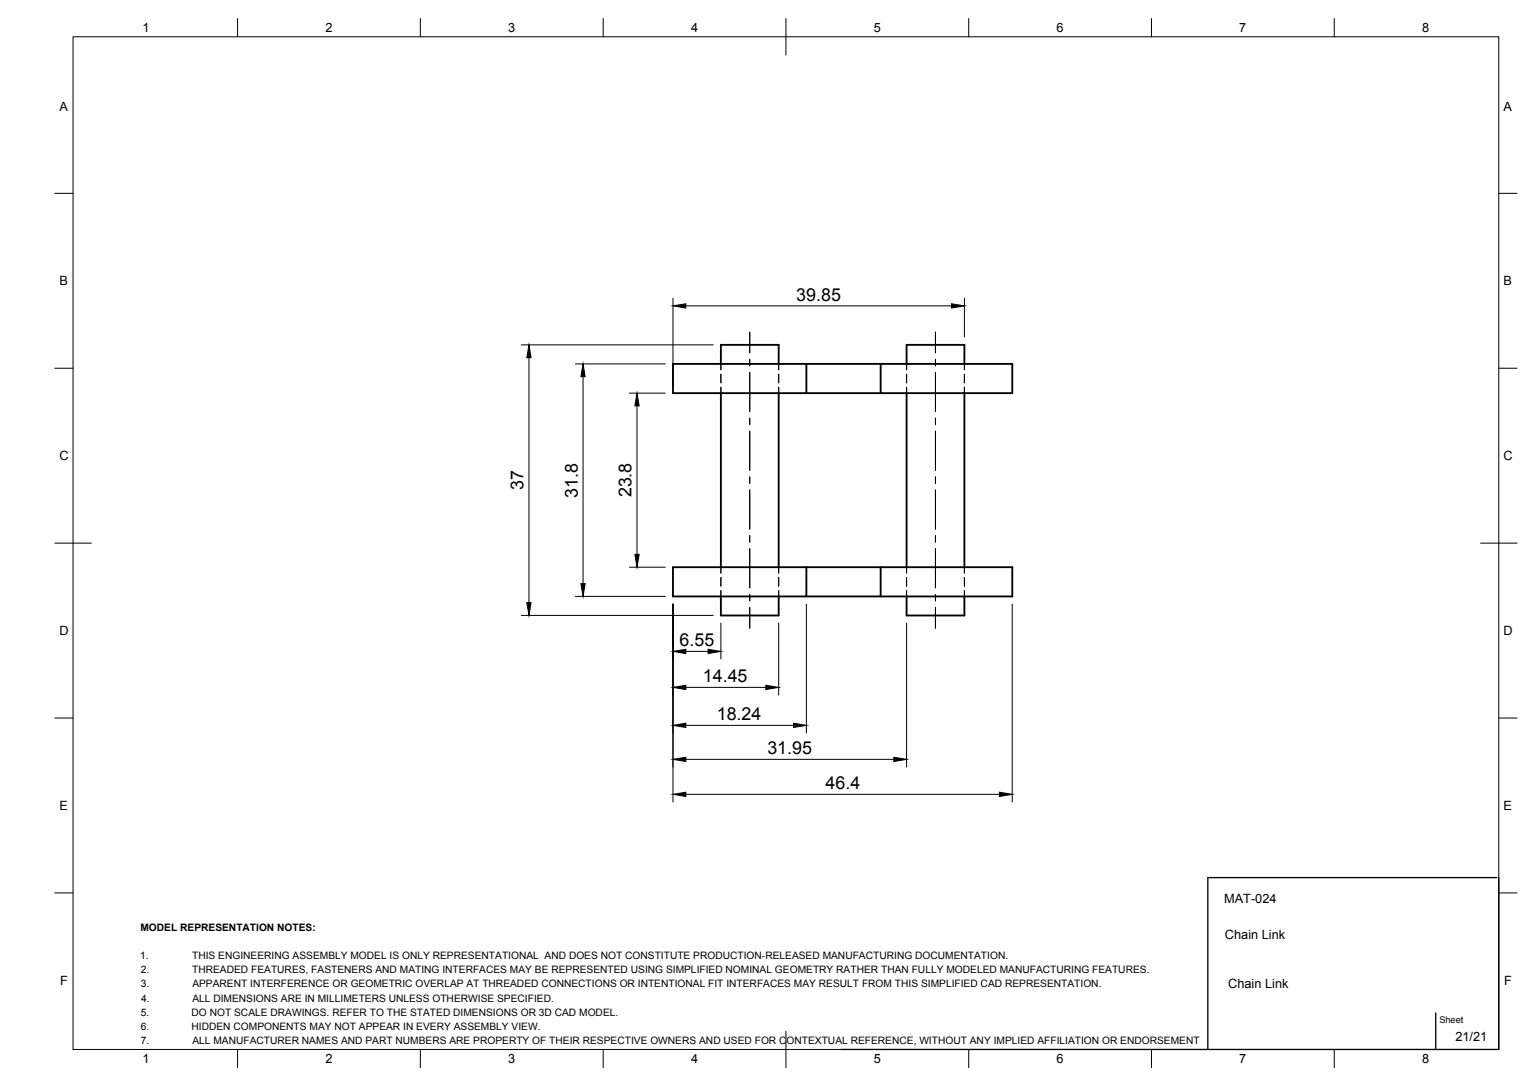
ISO-10303-21;
HEADER;
/* Generated by software containing ST-Developer
 * from STEP Tools, Inc. (www.steptools.com) 
 */

FILE_DESCRIPTION(
/* description */ ('STEP AP214'),
/* implementation_level */ '2;1');

FILE_NAME(
/* name */ 'Chain Link.step',
/* time_stamp */ '2026-11-14T06:34:07-08:00',
/* author */ (''),
/* organization */ (''),
/* preprocessor_version */ 'ST-DEVELOPER v20.2',
/* originating_system */ 'Autodesk Translation Framework v15.17.0.0',
/* authorisation */ '');

FILE_SCHEMA (('AUTOMOTIVE_DESIGN { 1 0 10303 214 3 1 1 }'));
ENDSEC;

DATA;
#10=MECHANICAL_DESIGN_GEOMETRIC_PRESENTATION_REPRESENTATION('',(#7282,#7283,#7284,#7285),#310623);
#7228=SHAPE_REPRESENTATION_RELATIONSHIP('SRR','None',#310901,#7245);
#7245=ADVANCED_BREP_SHAPE_REPRESENTATION('',(#7350,#7351,#7352,#7353),#310610);
#7282=STYLED_ITEM('',(#311007),#7350);
#7283=STYLED_ITEM('',(#311007),#7351);
#7284=STYLED_ITEM('',(#311007),#7352);
#7285=STYLED_ITEM('',(#311007),#7353);
#7350=MANIFOLD_SOLID_BREP('Body1',#93732);
#7351=MANIFOLD_SOLID_BREP('Body2',#93733);
#7352=MANIFOLD_SOLID_BREP('Body3',#93734);
#7353=MANIFOLD_SOLID_BREP('Body4',#93735);
#7630=FACE_BOUND('',#19915,.T.);
#7631=FACE_BOUND('',#19916,.T.);
#7632=FACE_BOUND('',#19918,.T.);
#7633=FACE_BOUND('',#19919,.T.);
#7634=FACE_BOUND('',#19924,.T.);
#7635=FACE_BOUND('',#19925,.T.);
#7636=FACE_BOUND('',#19927,.T.);
#7637=FACE_BOUND('',#19928,.T.);
#8541=PLANE('',#103942);
#8542=PLANE('',#103943);
#8543=PLANE('',#103953);
#8544=PLANE('',#103957);
#8545=PLANE('',#103967);
#8546=PLANE('',#103968);
#8547=PLANE('',#103972);
#8548=PLANE('',#103973);
#13930=FACE_OUTER_BOUND('',#19908,.T.);
#13931=FACE_OUTER_BOUND('',#19909,.T.);
#13932=FACE_OUTER_BOUND('',#19910,.T.);
#13933=FACE_OUTER_BOUND('',#19911,.T.);
#13934=FACE_OUTER_BOUND('',#19912,.T.);
#13935=FACE_OUTER_BOUND('',#19913,.T.);
#13936=FACE_OUTER_BOUND('',#19914,.T.);
#13937=FACE_OUTER_BOUND('',#19917,.T.);
#13938=FACE_OUTER_BOUND('',#19920,.T.);
#13939=FACE_OUTER_BOUND('',#19921,.T.);
#13940=FACE_OUTER_BOUND('',#19922,.T.);
#13941=FACE_OUTER_BOUND('',#19923,.T.);
#13942=FACE_OUTER_BOUND('',#19926,.T.);
#13943=FACE_OUTER_BOUND('',#19929,.T.);
#13944=FACE_OUTER_BOUND('',#19930,.T.);
#13945=FACE_OUTER_BOUND('',#19931,.T.);
#13946=FACE_OUTER_BOUND('',#19932,.T.);
#13947=FACE_OUTER_BOUND('',#19933,.T.);
#13948=FACE_OUTER_BOUND('',#19934,.T.);
#13949=FACE_OUTER_BOUND('',#19935,.T.);
#13950=FACE_OUTER_BOUND('',#19936,.T.);
#13951=FACE_OUTER_BOUND('',#19937,.T.);
#19908=EDGE_LOOP('',(#83435,#83436,#83437,#83438));
#19909=EDGE_LOOP('',(#83439,#83440,#83441,#83442));
#19910=EDGE_LOOP('',(#83443,#83444,#83445,#83446));
#19911=EDGE_LOOP('',(#83447,#83448,#83449,#83450));
#19912=EDGE_LOOP('',(#83451,#83452,#83453,#83454));
#19913=EDGE_LOOP('',(#83455,#83456,#83457,#83458));
#19914=EDGE_LOOP('',(#83459,#83460,#83461,#83462));
#19915=EDGE_LOOP('',(#83463));
#19916=EDGE_LOOP('',(#83464));
#19917=EDGE_LOOP('',(#83465,#83466,#83467,#83468));
#19918=EDGE_LOOP('',(#83469));
#19919=EDGE_LOOP('',(#83470));
#19920=EDGE_LOOP('',(#83471,#83472,#83473,#83474));
#19921=EDGE_LOOP('',(#83475,#83476,#83477,#83478));
#19922=EDGE_LOOP('',(#83479,#83480,#83481,#83482));
#19923=EDGE_LOOP('',(#83483,#83484,#83485,#83486));
#19924=EDGE_LOOP('',(#83487));
#19925=EDGE_LOOP('',(#83488));
#19926=EDGE_LOOP('',(#83489,#83490,#83491,#83492));
#19927=EDGE_LOOP('',(#83493));
#19928=EDGE_LOOP('',(#83494));
#19929=EDGE_LOOP('',(#83495,#83496,#83497,#83498));
#19930=EDGE_LOOP('',(#83499,#83500,#83501,#83502));
#19931=EDGE_LOOP('',(#83503,#83504,#83505,#83506));
#19932=EDGE_LOOP('',(#83507,#83508,#83509,#83510));
#19933=EDGE_LOOP('',(#83511));
#19934=EDGE_LOOP('',(#83512));
#19935=EDGE_LOOP('',(#83513,#83514,#83515,#83516));
#19936=EDGE_LOOP('',(#83517));
#19937=EDGE_LOOP('',(#83518));
#24417=LINE('',#275070,#28764);
#24418=LINE('',#275077,#28765);
#24419=LINE('',#275080,#28766);
#24420=LINE('',#275085,#28767);
#24421=LINE('',#275091,#28768);
#24422=LINE('',#275097,#28769);
#24423=LINE('',#275108,#28770);
#24424=LINE('',#275114,#28771);
#24425=LINE('',#275121,#28772);
#24426=LINE('',#275124,#28773);
#24427=LINE('',#275138,#28774);
#24428=LINE('',#275140,#28775);
#24429=LINE('',#275146,#28776);
#24430=LINE('',#275154,#28777);
#28764=VECTOR('',#128726,3.95);
#28765=VECTOR('',#128733,1000.);
#28766=VECTOR('',#128736,1000.);
#28767=VECTOR('',#128741,3.95);
#28768=VECTOR('',#128748,1000.);
#28769=VECTOR('',#128755,1000.);
#28770=VECTOR('',#128772,3.95);
#28771=VECTOR('',#128779,3.95);
#28772=VECTOR('',#128786,1000.);
#28773=VECTOR('',#128789,1000.);
#28774=VECTOR('',#128808,1000.);
#28775=VECTOR('',#128811,1000.);
#28776=VECTOR('',#128818,3.95);
#28777=VECTOR('',#128829,3.95);
#34851=CIRCLE('',#103925,3.95);
#34852=CIRCLE('',#103926,3.95);
#34853=CIRCLE('',#103928,10.5);
#34854=CIRCLE('',#103929,10.5);
#34855=CIRCLE('',#103931,3.95);
#34856=CIRCLE('',#103932,3.95);
#34857=CIRCLE('',#103934,10.5);
#34858=CIRCLE('',#103935,10.5);
#34859=CIRCLE('',#103937,10.5);
#34860=CIRCLE('',#103938,10.5);
#34861=CIRCLE('',#103940,10.5);
#34862=CIRCLE('',#103941,10.5);
#34863=CIRCLE('',#103945,3.95);
#34864=CIRCLE('',#103946,3.95);
#34865=CIRCLE('',#103948,3.95);
#34866=CIRCLE('',#103949,3.95);
#34867=CIRCLE('',#103951,10.5);
#34868=CIRCLE('',#103952,10.5);
#34869=CIRCLE('',#103954,10.5);
#34870=CIRCLE('',#103955,10.5);
#34871=CIRCLE('',#103956,10.5);
#34872=CIRCLE('',#103958,10.5);
#34873=CIRCLE('',#103959,10.5);
#34874=CIRCLE('',#103960,10.5);
#34875=CIRCLE('',#103965,3.95);
#34876=CIRCLE('',#103966,3.95);
#34877=CIRCLE('',#103970,3.95);
#34878=CIRCLE('',#103971,3.95);
#42825=VERTEX_POINT('',#275067);
#42826=VERTEX_POINT('',#275069);
#42827=VERTEX_POINT('',#275073);
#42828=VERTEX_POINT('',#275074);
#42829=VERTEX_POINT('',#275076);
#42830=VERTEX_POINT('',#275078);
#42831=VERTEX_POINT('',#275082);
#42832=VERTEX_POINT('',#275084);
#42833=VERTEX_POINT('',#275088);
#42834=VERTEX_POINT('',#275090);
#42835=VERTEX_POINT('',#275094);
#42836=VERTEX_POINT('',#275096);
#42837=VERTEX_POINT('',#275105);
#42838=VERTEX_POINT('',#275107);
#42839=VERTEX_POINT('',#275111);
#42840=VERTEX_POINT('',#275113);
#42841=VERTEX_POINT('',#275117);
#42842=VERTEX_POINT('',#275118);
#42843=VERTEX_POINT('',#275120);
#42844=VERTEX_POINT('',#275122);
#42845=VERTEX_POINT('',#275126);
#42846=VERTEX_POINT('',#275128);
#42847=VERTEX_POINT('',#275132);
#42848=VERTEX_POINT('',#275134);
#42849=VERTEX_POINT('',#275143);
#42850=VERTEX_POINT('',#275145);
#42851=VERTEX_POINT('',#275151);
#42852=VERTEX_POINT('',#275153);
#56497=EDGE_CURVE('',#42825,#42825,#34851,.T.);
#56498=EDGE_CURVE('',#42825,#42826,#24417,.T.);
#56499=EDGE_CURVE('',#42826,#42826,#34852,.T.);
#56500=EDGE_CURVE('',#42827,#42828,#34853,.T.);
#56501=EDGE_CURVE('',#42827,#42829,#24418,.T.);
#56502=EDGE_CURVE('',#42829,#42830,#34854,.T.);
#56503=EDGE_CURVE('',#42828,#42830,#24419,.T.);
#56504=EDGE_CURVE('',#42831,#42831,#34855,.T.);
#56505=EDGE_CURVE('',#42831,#42832,#24420,.T.);
#56506=EDGE_CURVE('',#42832,#42832,#34856,.T.);
#56507=EDGE_CURVE('',#42830,#42833,#34857,.T.);
#56508=EDGE_CURVE('',#42834,#42833,#24421,.T.);
#56509=EDGE_CURVE('',#42828,#42834,#34858,.T.);
#56510=EDGE_CURVE('',#42833,#42835,#34859,.T.);
#56511=EDGE_CURVE('',#42836,#42835,#24422,.T.);
#56512=EDGE_CURVE('',#42834,#42836,#34860,.T.);
#56513=EDGE_CURVE('',#42829,#42835,#34861,.T.);
#56514=EDGE_CURVE('',#42827,#42836,#34862,.T.);
#56515=EDGE_CURVE('',#42837,#42837,#34863,.T.);
#56516=EDGE_CURVE('',#42837,#42838,#24423,.T.);
#56517=EDGE_CURVE('',#42838,#42838,#34864,.T.);
#56518=EDGE_CURVE('',#42839,#42839,#34865,.T.);
#56519=EDGE_CURVE('',#42839,#42840,#24424,.T.);
#56520=EDGE_CURVE('',#42840,#42840,#34866,.T.);
#56521=EDGE_CURVE('',#42841,#42842,#34867,.T.);
#56522=EDGE_CURVE('',#42841,#42843,#24425,.T.);
#56523=EDGE_CURVE('',#42843,#42844,#34868,.T.);
#56524=EDGE_CURVE('',#42842,#42844,#24426,.T.);
#56525=EDGE_CURVE('',#42842,#42845,#34869,.T.);
#56526=EDGE_CURVE('',#42845,#42846,#34870,.T.);
#56527=EDGE_CURVE('',#42846,#42841,#34871,.T.);
#56528=EDGE_CURVE('',#42844,#42847,#34872,.T.);
#56529=EDGE_CURVE('',#42848,#42843,#34873,.T.);
#56530=EDGE_CURVE('',#42847,#42848,#34874,.T.);
#56531=EDGE_CURVE('',#42845,#42847,#24427,.T.);
#56532=EDGE_CURVE('',#42846,#42848,#24428,.T.);
#56533=EDGE_CURVE('',#42849,#42849,#34875,.T.);
#56534=EDGE_CURVE('',#42849,#42850,#24429,.T.);
#56535=EDGE_CURVE('',#42850,#42850,#34876,.T.);
#56536=EDGE_CURVE('',#42851,#42851,#34877,.T.);
#56537=EDGE_CURVE('',#42851,#42852,#24430,.T.);
#56538=EDGE_CURVE('',#42852,#42852,#34878,.T.);
#83435=ORIENTED_EDGE('',*,*,#56497,.T.);
#83436=ORIENTED_EDGE('',*,*,#56498,.T.);
#83437=ORIENTED_EDGE('',*,*,#56499,.F.);
#83438=ORIENTED_EDGE('',*,*,#56498,.F.);
#83439=ORIENTED_EDGE('',*,*,#56500,.F.);
#83440=ORIENTED_EDGE('',*,*,#56501,.T.);
#83441=ORIENTED_EDGE('',*,*,#56502,.T.);
#83442=ORIENTED_EDGE('',*,*,#56503,.F.);
#83443=ORIENTED_EDGE('',*,*,#56504,.T.);
#83444=ORIENTED_EDGE('',*,*,#56505,.T.);
#83445=ORIENTED_EDGE('',*,*,#56506,.F.);
#83446=ORIENTED_EDGE('',*,*,#56505,.F.);
#83447=ORIENTED_EDGE('',*,*,#56507,.T.);
#83448=ORIENTED_EDGE('',*,*,#56508,.F.);
#83449=ORIENTED_EDGE('',*,*,#56509,.F.);
#83450=ORIENTED_EDGE('',*,*,#56503,.T.);
#83451=ORIENTED_EDGE('',*,*,#56510,.T.);
#83452=ORIENTED_EDGE('',*,*,#56511,.F.);
#83453=ORIENTED_EDGE('',*,*,#56512,.F.);
#83454=ORIENTED_EDGE('',*,*,#56508,.T.);
#83455=ORIENTED_EDGE('',*,*,#56513,.F.);
#83456=ORIENTED_EDGE('',*,*,#56501,.F.);
#83457=ORIENTED_EDGE('',*,*,#56514,.T.);
#83458=ORIENTED_EDGE('',*,*,#56511,.T.);
#83459=ORIENTED_EDGE('',*,*,#56509,.T.);
#83460=ORIENTED_EDGE('',*,*,#56512,.T.);
#83461=ORIENTED_EDGE('',*,*,#56514,.F.);
#83462=ORIENTED_EDGE('',*,*,#56500,.T.);
#83463=ORIENTED_EDGE('',*,*,#56504,.F.);
#83464=ORIENTED_EDGE('',*,*,#56497,.F.);
#83465=ORIENTED_EDGE('',*,*,#56507,.F.);
#83466=ORIENTED_EDGE('',*,*,#56502,.F.);
#83467=ORIENTED_EDGE('',*,*,#56513,.T.);
#83468=ORIENTED_EDGE('',*,*,#56510,.F.);
#83469=ORIENTED_EDGE('',*,*,#56506,.T.);
#83470=ORIENTED_EDGE('',*,*,#56499,.T.);
#83471=ORIENTED_EDGE('',*,*,#56515,.T.);
#83472=ORIENTED_EDGE('',*,*,#56516,.T.);
#83473=ORIENTED_EDGE('',*,*,#56517,.F.);
#83474=ORIENTED_EDGE('',*,*,#56516,.F.);
#83475=ORIENTED_EDGE('',*,*,#56518,.T.);
#83476=ORIENTED_EDGE('',*,*,#56519,.T.);
#83477=ORIENTED_EDGE('',*,*,#56520,.F.);
#83478=ORIENTED_EDGE('',*,*,#56519,.F.);
#83479=ORIENTED_EDGE('',*,*,#56521,.F.);
#83480=ORIENTED_EDGE('',*,*,#56522,.T.);
#83481=ORIENTED_EDGE('',*,*,#56523,.T.);
#83482=ORIENTED_EDGE('',*,*,#56524,.F.);
#83483=ORIENTED_EDGE('',*,*,#56525,.T.);
#83484=ORIENTED_EDGE('',*,*,#56526,.T.);
#83485=ORIENTED_EDGE('',*,*,#56527,.T.);
#83486=ORIENTED_EDGE('',*,*,#56521,.T.);
#83487=ORIENTED_EDGE('',*,*,#56515,.F.);
#83488=ORIENTED_EDGE('',*,*,#56518,.F.);
#83489=ORIENTED_EDGE('',*,*,#56528,.F.);
#83490=ORIENTED_EDGE('',*,*,#56523,.F.);
#83491=ORIENTED_EDGE('',*,*,#56529,.F.);
#83492=ORIENTED_EDGE('',*,*,#56530,.F.);
#83493=ORIENTED_EDGE('',*,*,#56520,.T.);
#83494=ORIENTED_EDGE('',*,*,#56517,.T.);
#83495=ORIENTED_EDGE('',*,*,#56528,.T.);
#83496=ORIENTED_EDGE('',*,*,#56531,.F.);
#83497=ORIENTED_EDGE('',*,*,#56525,.F.);
#83498=ORIENTED_EDGE('',*,*,#56524,.T.);
#83499=ORIENTED_EDGE('',*,*,#56530,.T.);
#83500=ORIENTED_EDGE('',*,*,#56532,.F.);
#83501=ORIENTED_EDGE('',*,*,#56526,.F.);
#83502=ORIENTED_EDGE('',*,*,#56531,.T.);
#83503=ORIENTED_EDGE('',*,*,#56529,.T.);
#83504=ORIENTED_EDGE('',*,*,#56522,.F.);
#83505=ORIENTED_EDGE('',*,*,#56527,.F.);
#83506=ORIENTED_EDGE('',*,*,#56532,.T.);
#83507=ORIENTED_EDGE('',*,*,#56533,.T.);
#83508=ORIENTED_EDGE('',*,*,#56534,.T.);
#83509=ORIENTED_EDGE('',*,*,#56535,.F.);
#83510=ORIENTED_EDGE('',*,*,#56534,.F.);
#83511=ORIENTED_EDGE('',*,*,#56535,.T.);
#83512=ORIENTED_EDGE('',*,*,#56533,.F.);
#83513=ORIENTED_EDGE('',*,*,#56536,.T.);
#83514=ORIENTED_EDGE('',*,*,#56537,.T.);
#83515=ORIENTED_EDGE('',*,*,#56538,.F.);
#83516=ORIENTED_EDGE('',*,*,#56537,.F.);
#83517=ORIENTED_EDGE('',*,*,#56538,.T.);
#83518=ORIENTED_EDGE('',*,*,#56536,.F.);
#87761=CYLINDRICAL_SURFACE('',#103924,3.95);
#87762=CYLINDRICAL_SURFACE('',#103927,10.5);
#87763=CYLINDRICAL_SURFACE('',#103930,3.95);
#87764=CYLINDRICAL_SURFACE('',#103933,10.5);
#87765=CYLINDRICAL_SURFACE('',#103936,10.5);
#87766=CYLINDRICAL_SURFACE('',#103939,10.5);
#87767=CYLINDRICAL_SURFACE('',#103944,3.95);
#87768=CYLINDRICAL_SURFACE('',#103947,3.95);
#87769=CYLINDRICAL_SURFACE('',#103950,10.5);
#87770=CYLINDRICAL_SURFACE('',#103961,10.5);
#87771=CYLINDRICAL_SURFACE('',#103962,10.5);
#87772=CYLINDRICAL_SURFACE('',#103963,10.5);
#87773=CYLINDRICAL_SURFACE('',#103964,3.95);
#87774=CYLINDRICAL_SURFACE('',#103969,3.95);
#93209=ADVANCED_FACE('',(#13930),#87761,.F.);
#93210=ADVANCED_FACE('',(#13931),#87762,.T.);
#93211=ADVANCED_FACE('',(#13932),#87763,.F.);
#93212=ADVANCED_FACE('',(#13933),#87764,.F.);
#93213=ADVANCED_FACE('',(#13934),#87765,.T.);
#93214=ADVANCED_FACE('',(#13935),#87766,.F.);
#93215=ADVANCED_FACE('',(#13936,#7630,#7631),#8541,.T.);
#93216=ADVANCED_FACE('',(#13937,#7632,#7633),#8542,.F.);
#93217=ADVANCED_FACE('',(#13938),#87767,.F.);
#93218=ADVANCED_FACE('',(#13939),#87768,.F.);
#93219=ADVANCED_FACE('',(#13940),#87769,.T.);
#93220=ADVANCED_FACE('',(#13941,#7634,#7635),#8543,.T.);
#93221=ADVANCED_FACE('',(#13942,#7636,#7637),#8544,.F.);
#93222=ADVANCED_FACE('',(#13943),#87770,.F.);
#93223=ADVANCED_FACE('',(#13944),#87771,.T.);
#93224=ADVANCED_FACE('',(#13945),#87772,.F.);
#93225=ADVANCED_FACE('',(#13946),#87773,.T.);
#93226=ADVANCED_FACE('',(#13947),#8545,.T.);
#93227=ADVANCED_FACE('',(#13948),#8546,.F.);
#93228=ADVANCED_FACE('',(#13949),#87774,.T.);
#93229=ADVANCED_FACE('',(#13950),#8547,.T.);
#93230=ADVANCED_FACE('',(#13951),#8548,.F.);
#93732=CLOSED_SHELL('',(#93209,#93210,#93211,#93212,#93213,#93214,#93215,
#93216));
#93733=CLOSED_SHELL('',(#93217,#93218,#93219,#93220,#93221,#93222,#93223,
#93224));
#93734=CLOSED_SHELL('',(#93225,#93226,#93227));
#93735=CLOSED_SHELL('',(#93228,#93229,#93230));
#103923=AXIS2_PLACEMENT_3D('',#275065,#128720,#128721);
#103924=AXIS2_PLACEMENT_3D('',#275066,#128722,#128723);
#103925=AXIS2_PLACEMENT_3D('',#275068,#128724,#128725);
#103926=AXIS2_PLACEMENT_3D('',#275071,#128727,#128728);
#103927=AXIS2_PLACEMENT_3D('',#275072,#128729,#128730);
#103928=AXIS2_PLACEMENT_3D('',#275075,#128731,#128732);
#103929=AXIS2_PLACEMENT_3D('',#275079,#128734,#128735);
#103930=AXIS2_PLACEMENT_3D('',#275081,#128737,#128738);
#103931=AXIS2_PLACEMENT_3D('',#275083,#128739,#128740);
#103932=AXIS2_PLACEMENT_3D('',#275086,#128742,#128743);
#103933=AXIS2_PLACEMENT_3D('',#275087,#128744,#128745);
#103934=AXIS2_PLACEMENT_3D('',#275089,#128746,#128747);
#103935=AXIS2_PLACEMENT_3D('',#275092,#128749,#128750);
#103936=AXIS2_PLACEMENT_3D('',#275093,#128751,#128752);
#103937=AXIS2_PLACEMENT_3D('',#275095,#128753,#128754);
#103938=AXIS2_PLACEMENT_3D('',#275098,#128756,#128757);
#103939=AXIS2_PLACEMENT_3D('',#275099,#128758,#128759);
#103940=AXIS2_PLACEMENT_3D('',#275100,#128760,#128761);
#103941=AXIS2_PLACEMENT_3D('',#275101,#128762,#128763);
#103942=AXIS2_PLACEMENT_3D('',#275102,#128764,#128765);
#103943=AXIS2_PLACEMENT_3D('',#275103,#128766,#128767);
#103944=AXIS2_PLACEMENT_3D('',#275104,#128768,#128769);
#103945=AXIS2_PLACEMENT_3D('',#275106,#128770,#128771);
#103946=AXIS2_PLACEMENT_3D('',#275109,#128773,#128774);
#103947=AXIS2_PLACEMENT_3D('',#275110,#128775,#128776);
#103948=AXIS2_PLACEMENT_3D('',#275112,#128777,#128778);
#103949=AXIS2_PLACEMENT_3D('',#275115,#128780,#128781);
#103950=AXIS2_PLACEMENT_3D('',#275116,#128782,#128783);
#103951=AXIS2_PLACEMENT_3D('',#275119,#128784,#128785);
#103952=AXIS2_PLACEMENT_3D('',#275123,#128787,#128788);
#103953=AXIS2_PLACEMENT_3D('',#275125,#128790,#128791);
#103954=AXIS2_PLACEMENT_3D('',#275127,#128792,#128793);
#103955=AXIS2_PLACEMENT_3D('',#275129,#128794,#128795);
#103956=AXIS2_PLACEMENT_3D('',#275130,#128796,#128797);
#103957=AXIS2_PLACEMENT_3D('',#275131,#128798,#128799);
#103958=AXIS2_PLACEMENT_3D('',#275133,#128800,#128801);
#103959=AXIS2_PLACEMENT_3D('',#275135,#128802,#128803);
#103960=AXIS2_PLACEMENT_3D('',#275136,#128804,#128805);
#103961=AXIS2_PLACEMENT_3D('',#275137,#128806,#128807);
#103962=AXIS2_PLACEMENT_3D('',#275139,#128809,#128810);
#103963=AXIS2_PLACEMENT_3D('',#275141,#128812,#128813);
#103964=AXIS2_PLACEMENT_3D('',#275142,#128814,#128815);
#103965=AXIS2_PLACEMENT_3D('',#275144,#128816,#128817);
#103966=AXIS2_PLACEMENT_3D('',#275147,#128819,#128820);
#103967=AXIS2_PLACEMENT_3D('',#275148,#128821,#128822);
#103968=AXIS2_PLACEMENT_3D('',#275149,#128823,#128824);
#103969=AXIS2_PLACEMENT_3D('',#275150,#128825,#128826);
#103970=AXIS2_PLACEMENT_3D('',#275152,#128827,#128828);
#103971=AXIS2_PLACEMENT_3D('',#275155,#128830,#128831);
#103972=AXIS2_PLACEMENT_3D('',#275156,#128832,#128833);
#103973=AXIS2_PLACEMENT_3D('',#275157,#128834,#128835);
#128720=DIRECTION('axis',(0.,0.,1.));
#128721=DIRECTION('refdir',(1.,0.,0.));
#128722=DIRECTION('center_axis',(0.,0.,-1.));
#128723=DIRECTION('ref_axis',(-1.,0.,0.));
#128724=DIRECTION('center_axis',(0.,0.,1.));
#128725=DIRECTION('ref_axis',(1.,0.,0.));
#128726=DIRECTION('',(0.,0.,-1.));
#128727=DIRECTION('center_axis',(0.,0.,1.));
#128728=DIRECTION('ref_axis',(1.,0.,0.));
#128729=DIRECTION('center_axis',(0.,0.,-1.));
#128730=DIRECTION('ref_axis',(-1.,0.,0.));
#128731=DIRECTION('center_axis',(0.,0.,1.));
#128732=DIRECTION('ref_axis',(1.,0.,0.));
#128733=DIRECTION('',(0.,0.,-1.));
#128734=DIRECTION('center_axis',(0.,0.,1.));
#128735=DIRECTION('ref_axis',(1.,0.,0.));
#128736=DIRECTION('',(0.,0.,-1.));
#128737=DIRECTION('center_axis',(0.,0.,-1.));
#128738=DIRECTION('ref_axis',(-1.,0.,0.));
#128739=DIRECTION('center_axis',(0.,0.,1.));
#128740=DIRECTION('ref_axis',(1.,0.,0.));
#128741=DIRECTION('',(0.,0.,-1.));
#128742=DIRECTION('center_axis',(0.,0.,1.));
#128743=DIRECTION('ref_axis',(1.,0.,0.));
#128744=DIRECTION('center_axis',(0.,0.,-1.));
#128745=DIRECTION('ref_axis',(-1.,0.,0.));
#128746=DIRECTION('center_axis',(0.,0.,-1.));
#128747=DIRECTION('ref_axis',(1.,0.,0.));
#128748=DIRECTION('',(0.,0.,-1.));
#128749=DIRECTION('center_axis',(0.,0.,-1.));
#128750=DIRECTION('ref_axis',(1.,0.,0.));
#128751=DIRECTION('center_axis',(0.,0.,-1.));
#128752=DIRECTION('ref_axis',(1.,1.22464679914735E-16,0.));
#128753=DIRECTION('center_axis',(0.,0.,1.));
#128754=DIRECTION('ref_axis',(1.,0.,0.));
#128755=DIRECTION('',(0.,0.,-1.));
#128756=DIRECTION('center_axis',(0.,0.,1.));
#128757=DIRECTION('ref_axis',(1.,0.,0.));
#128758=DIRECTION('center_axis',(0.,0.,-1.));
#128759=DIRECTION('ref_axis',(-1.,0.,0.));
#128760=DIRECTION('center_axis',(0.,0.,1.));
#128761=DIRECTION('ref_axis',(1.,0.,0.));
#128762=DIRECTION('center_axis',(0.,0.,1.));
#128763=DIRECTION('ref_axis',(1.,0.,0.));
#128764=DIRECTION('center_axis',(0.,0.,1.));
#128765=DIRECTION('ref_axis',(1.,0.,0.));
#128766=DIRECTION('center_axis',(0.,0.,1.));
#128767=DIRECTION('ref_axis',(1.,0.,0.));
#128768=DIRECTION('center_axis',(0.,0.,-1.));
#128769=DIRECTION('ref_axis',(-1.,0.,0.));
#128770=DIRECTION('center_axis',(0.,0.,1.));
#128771=DIRECTION('ref_axis',(1.,0.,0.));
#128772=DIRECTION('',(0.,0.,-1.));
#128773=DIRECTION('center_axis',(0.,0.,1.));
#128774=DIRECTION('ref_axis',(1.,0.,0.));
#128775=DIRECTION('center_axis',(0.,0.,-1.));
#128776=DIRECTION('ref_axis',(-1.,0.,0.));
#128777=DIRECTION('center_axis',(0.,0.,1.));
#128778=DIRECTION('ref_axis',(1.,0.,0.));
#128779=DIRECTION('',(0.,0.,-1.));
#128780=DIRECTION('center_axis',(0.,0.,1.));
#128781=DIRECTION('ref_axis',(1.,0.,0.));
#128782=DIRECTION('center_axis',(0.,0.,-1.));
#128783=DIRECTION('ref_axis',(-1.,0.,0.));
#128784=DIRECTION('center_axis',(0.,0.,1.));
#128785=DIRECTION('ref_axis',(1.,0.,0.));
#128786=DIRECTION('',(0.,0.,-1.));
#128787=DIRECTION('center_axis',(0.,0.,1.));
#128788=DIRECTION('ref_axis',(1.,0.,0.));
#128789=DIRECTION('',(0.,0.,-1.));
#128790=DIRECTION('center_axis',(0.,0.,1.));
#128791=DIRECTION('ref_axis',(1.,0.,0.));
#128792=DIRECTION('center_axis',(0.,0.,-1.));
#128793=DIRECTION('ref_axis',(1.,0.,0.));
#128794=DIRECTION('center_axis',(0.,0.,1.));
#128795=DIRECTION('ref_axis',(1.,0.,0.));
#128796=DIRECTION('center_axis',(0.,0.,-1.));
#128797=DIRECTION('ref_axis',(1.,0.,0.));
#128798=DIRECTION('center_axis',(0.,0.,1.));
#128799=DIRECTION('ref_axis',(1.,0.,0.));
#128800=DIRECTION('center_axis',(0.,0.,-1.));
#128801=DIRECTION('ref_axis',(1.,0.,0.));
#128802=DIRECTION('center_axis',(0.,0.,-1.));
#128803=DIRECTION('ref_axis',(1.,0.,0.));
#128804=DIRECTION('center_axis',(0.,0.,1.));
#128805=DIRECTION('ref_axis',(1.,0.,0.));
#128806=DIRECTION('center_axis',(0.,0.,-1.));
#128807=DIRECTION('ref_axis',(-1.,0.,0.));
#128808=DIRECTION('',(0.,0.,-1.));
#128809=DIRECTION('center_axis',(0.,0.,-1.));
#128810=DIRECTION('ref_axis',(1.,-3.21624529935327E-16,0.));
#128811=DIRECTION('',(0.,0.,-1.));
#128812=DIRECTION('center_axis',(0.,0.,-1.));
#128813=DIRECTION('ref_axis',(-1.,0.,0.));
#128814=DIRECTION('center_axis',(0.,0.,-1.));
#128815=DIRECTION('ref_axis',(-1.,0.,0.));
#128816=DIRECTION('center_axis',(0.,0.,1.));
#128817=DIRECTION('ref_axis',(1.,0.,0.));
#128818=DIRECTION('',(0.,0.,1.));
#128819=DIRECTION('center_axis',(0.,0.,1.));
#128820=DIRECTION('ref_axis',(1.,0.,0.));
#128821=DIRECTION('center_axis',(0.,0.,1.));
#128822=DIRECTION('ref_axis',(1.,0.,0.));
#128823=DIRECTION('center_axis',(0.,0.,1.));
#128824=DIRECTION('ref_axis',(1.,0.,0.));
#128825=DIRECTION('center_axis',(0.,0.,-1.));
#128826=DIRECTION('ref_axis',(-1.,0.,0.));
#128827=DIRECTION('center_axis',(0.,0.,1.));
#128828=DIRECTION('ref_axis',(1.,0.,0.));
#128829=DIRECTION('',(0.,0.,1.));
#128830=DIRECTION('center_axis',(0.,0.,1.));
#128831=DIRECTION('ref_axis',(1.,0.,0.));
#128832=DIRECTION('center_axis',(0.,0.,1.));
#128833=DIRECTION('ref_axis',(1.,0.,0.));
#128834=DIRECTION('center_axis',(0.,0.,1.));
#128835=DIRECTION('ref_axis',(1.,0.,0.));
#275065=CARTESIAN_POINT('',(0.,0.,0.));
#275066=CARTESIAN_POINT('Origin',(12.6996622584713,0.0926203042559918,2.));
#275067=CARTESIAN_POINT('',(16.6496622584713,0.0926203042559914,2.));
#275068=CARTESIAN_POINT('Origin',(12.6996622584713,0.0926203042559918,2.));
#275069=CARTESIAN_POINT('',(16.6496622584713,0.0926203042559914,-2.));
#275070=CARTESIAN_POINT('',(16.6496622584713,0.0926203042559914,2.));
#275071=CARTESIAN_POINT('Origin',(12.6996622584713,0.0926203042559918,-2.));
#275072=CARTESIAN_POINT('Origin',(-12.7003377415287,0.0926203042559918,
2.));
#275073=CARTESIAN_POINT('',(-4.95988141030959,7.18736031249375,2.));
#275074=CARTESIAN_POINT('',(-4.9598814103096,-7.00211970398177,2.));
#275075=CARTESIAN_POINT('Origin',(-12.7003377415287,0.0926203042559918,
2.));
#275076=CARTESIAN_POINT('',(-4.95988141030959,7.18736031249375,-2.));
#275077=CARTESIAN_POINT('',(-4.95988141030959,7.18736031249375,2.));
#275078=CARTESIAN_POINT('',(-4.9598814103096,-7.00211970398177,-2.));
#275079=CARTESIAN_POINT('Origin',(-12.7003377415287,0.0926203042559918,
-2.));
#275080=CARTESIAN_POINT('',(-4.9598814103096,-7.00211970398177,2.));
#275081=CARTESIAN_POINT('Origin',(-12.7003377415287,0.0926203042559918,
2.));
#275082=CARTESIAN_POINT('',(-8.75033774152873,0.0926203042559914,2.));
#275083=CARTESIAN_POINT('Origin',(-12.7003377415287,0.0926203042559918,
2.));
#275084=CARTESIAN_POINT('',(-8.75033774152873,0.0926203042559914,-2.));
#275085=CARTESIAN_POINT('',(-8.75033774152873,0.0926203042559914,2.));
#275086=CARTESIAN_POINT('Origin',(-12.7003377415287,0.0926203042559918,
-2.));
#275087=CARTESIAN_POINT('Origin',(-0.10965027657137,-16.314759391488,2.));
#275088=CARTESIAN_POINT('',(5.20000000000002,-7.25619361425234,-2.));
#275089=CARTESIAN_POINT('Origin',(-0.10965027657137,-16.314759391488,-2.));
#275090=CARTESIAN_POINT('',(5.20000000000002,-7.25619361425234,2.));
#275091=CARTESIAN_POINT('',(5.20000000000002,-7.25619361425234,2.));
#275092=CARTESIAN_POINT('Origin',(-0.10965027657137,-16.314759391488,2.));
#275093=CARTESIAN_POINT('Origin',(12.6996622584713,0.0926203042559918,2.));
#275094=CARTESIAN_POINT('',(5.20000000000002,7.44143422276433,-2.));
#275095=CARTESIAN_POINT('Origin',(12.6996622584713,0.0926203042559918,-2.));
#275096=CARTESIAN_POINT('',(5.20000000000002,7.44143422276433,2.));
#275097=CARTESIAN_POINT('',(5.20000000000002,7.44143422276433,2.));
#275098=CARTESIAN_POINT('Origin',(12.6996622584713,0.0926203042559918,2.));
#275099=CARTESIAN_POINT('Origin',(-0.10965027657137,16.5,2.));
#275100=CARTESIAN_POINT('Origin',(-0.10965027657137,16.5,-2.));
#275101=CARTESIAN_POINT('Origin',(-0.10965027657137,16.5,2.));
#275102=CARTESIAN_POINT('Origin',(0.,0.,2.));
#275103=CARTESIAN_POINT('Origin',(0.,0.,-2.));
#275104=CARTESIAN_POINT('Origin',(-12.7003377415287,0.0926203042559918,
29.8));
#275105=CARTESIAN_POINT('',(-8.75033774152873,0.0926203042559914,29.8));
#275106=CARTESIAN_POINT('Origin',(-12.7003377415287,0.0926203042559918,
29.8));
#275107=CARTESIAN_POINT('',(-8.75033774152873,0.0926203042559914,25.8));
#275108=CARTESIAN_POINT('',(-8.75033774152873,0.0926203042559914,29.8));
#275109=CARTESIAN_POINT('Origin',(-12.7003377415287,0.0926203042559918,
25.8));
#275110=CARTESIAN_POINT('Origin',(12.6996622584713,0.0926203042559918,29.8));
#275111=CARTESIAN_POINT('',(16.6496622584713,0.0926203042559914,29.8));
#275112=CARTESIAN_POINT('Origin',(12.6996622584713,0.0926203042559918,29.8));
#275113=CARTESIAN_POINT('',(16.6496622584713,0.0926203042559914,25.8));
#275114=CARTESIAN_POINT('',(16.6496622584713,0.0926203042559914,29.8));
#275115=CARTESIAN_POINT('Origin',(12.6996622584713,0.0926203042559918,25.8));
#275116=CARTESIAN_POINT('Origin',(-12.7003377415287,0.0926203042559918,
29.8));
#275117=CARTESIAN_POINT('',(-4.9598814103096,7.18736031249375,29.8));
#275118=CARTESIAN_POINT('',(-4.9598814103096,-7.00211970398178,29.8));
#275119=CARTESIAN_POINT('Origin',(-12.7003377415287,0.0926203042559918,
29.8));
#275120=CARTESIAN_POINT('',(-4.9598814103096,7.18736031249375,25.8));
#275121=CARTESIAN_POINT('',(-4.9598814103096,7.18736031249375,29.8));
#275122=CARTESIAN_POINT('',(-4.9598814103096,-7.00211970398178,25.8));
#275123=CARTESIAN_POINT('Origin',(-12.7003377415287,0.0926203042559918,
25.8));
#275124=CARTESIAN_POINT('',(-4.9598814103096,-7.00211970398178,29.8));
#275125=CARTESIAN_POINT('Origin',(-6.40499400905005,-8.11106954361601,29.8));
#275126=CARTESIAN_POINT('',(5.20000000000001,-7.25619361425234,29.8));
#275127=CARTESIAN_POINT('Origin',(-0.10965027657137,-16.314759391488,29.8));
#275128=CARTESIAN_POINT('',(5.20000000000002,7.44143422276433,29.8));
#275129=CARTESIAN_POINT('Origin',(12.6996622584713,0.0926203042559918,29.8));
#275130=CARTESIAN_POINT('Origin',(-0.10965027657137,16.5,29.8));
#275131=CARTESIAN_POINT('Origin',(-6.40499400905005,-8.11106954361601,25.8));
#275132=CARTESIAN_POINT('',(5.20000000000001,-7.25619361425234,25.8));
#275133=CARTESIAN_POINT('Origin',(-0.10965027657137,-16.314759391488,25.8));
#275134=CARTESIAN_POINT('',(5.20000000000002,7.44143422276433,25.8));
#275135=CARTESIAN_POINT('Origin',(-0.10965027657137,16.5,25.8));
#275136=CARTESIAN_POINT('Origin',(12.6996622584713,0.0926203042559918,25.8));
#275137=CARTESIAN_POINT('Origin',(-0.10965027657137,-16.314759391488,29.8));
#275138=CARTESIAN_POINT('',(5.20000000000001,-7.25619361425234,29.8));
#275139=CARTESIAN_POINT('Origin',(12.6996622584713,0.0926203042559918,29.8));
#275140=CARTESIAN_POINT('',(5.20000000000002,7.44143422276433,29.8));
#275141=CARTESIAN_POINT('Origin',(-0.10965027657137,16.5,29.8));
#275142=CARTESIAN_POINT('Origin',(-12.7003377415287,0.0926203042559918,
32.4));
#275143=CARTESIAN_POINT('',(-8.75033774152873,0.0926203042559914,-4.59999999999999));
#275144=CARTESIAN_POINT('Origin',(-12.7003377415287,0.0926203042559918,
-4.6));
#275145=CARTESIAN_POINT('',(-8.75033774152873,0.0926203042559914,32.4));
#275146=CARTESIAN_POINT('',(-8.75033774152873,0.0926203042559914,32.4));
#275147=CARTESIAN_POINT('Origin',(-12.7003377415287,0.0926203042559918,
32.4));
#275148=CARTESIAN_POINT('Origin',(-12.7003377415287,0.0926203042559918,
32.4));
#275149=CARTESIAN_POINT('Origin',(-12.7003377415287,0.0926203042559918,
-4.6));
#275150=CARTESIAN_POINT('Origin',(12.6996622584713,0.0926203042559918,32.4));
#275151=CARTESIAN_POINT('',(16.6496622584713,0.0926203042559914,-4.59999999999999));
#275152=CARTESIAN_POINT('Origin',(12.6996622584713,0.0926203042559918,-4.6));
#275153=CARTESIAN_POINT('',(16.6496622584713,0.0926203042559914,32.4));
#275154=CARTESIAN_POINT('',(16.6496622584713,0.0926203042559914,32.4));
#275155=CARTESIAN_POINT('Origin',(12.6996622584713,0.0926203042559918,32.4));
#275156=CARTESIAN_POINT('Origin',(12.6996622584713,0.0926203042559918,32.4));
#275157=CARTESIAN_POINT('Origin',(12.6996622584713,0.0926203042559918,-4.6));
#310588=UNCERTAINTY_MEASURE_WITH_UNIT(LENGTH_MEASURE(0.01),#310624,
'DISTANCE_ACCURACY_VALUE',
'Maximum model space distance between geometric entities at asserted c
onnectivities');
#310601=UNCERTAINTY_MEASURE_WITH_UNIT(LENGTH_MEASURE(0.01),#310624,
'DISTANCE_ACCURACY_VALUE',
'Maximum model space distance between geometric entities at asserted c
onnectivities');
#310610=(
GEOMETRIC_REPRESENTATION_CONTEXT(3)
GLOBAL_UNCERTAINTY_ASSIGNED_CONTEXT((#310588))
GLOBAL_UNIT_ASSIGNED_CONTEXT((#310624,#310626,#310627))
REPRESENTATION_CONTEXT('','3D')
);
#310623=(
GEOMETRIC_REPRESENTATION_CONTEXT(3)
GLOBAL_UNCERTAINTY_ASSIGNED_CONTEXT((#310601))
GLOBAL_UNIT_ASSIGNED_CONTEXT((#310624,#310626,#310627))
REPRESENTATION_CONTEXT('','3D')
);
#310624=(
LENGTH_UNIT()
NAMED_UNIT(*)
SI_UNIT(.MILLI.,.METRE.)
);
#310626=(
NAMED_UNIT(*)
PLANE_ANGLE_UNIT()
SI_UNIT($,.RADIAN.)
);
#310627=(
NAMED_UNIT(*)
SI_UNIT($,.STERADIAN.)
SOLID_ANGLE_UNIT()
);
#310636=SHAPE_DEFINITION_REPRESENTATION(#310657,#310901);
#310657=PRODUCT_DEFINITION_SHAPE('',$,#310923);
#310901=SHAPE_REPRESENTATION('',(#103923),#310610);
#310914=PRODUCT_DEFINITION_CONTEXT('part definition',#310979,'design');
#310923=PRODUCT_DEFINITION('Chain Link','Chain Link',#310944,#310914);
#310944=PRODUCT_DEFINITION_FORMATION('',$,#310989);
#310979=APPLICATION_CONTEXT(
'Core Data for Automotive Mechanical Design Process');
#310980=PRODUCT_CONTEXT('part definition',#310979,'mechanical');
#310989=PRODUCT('Chain Link','Chain Link',$,(#310980));
#311007=PRESENTATION_STYLE_ASSIGNMENT((#311014));
#311014=SURFACE_STYLE_USAGE(.BOTH.,#311021);
#311021=SURFACE_SIDE_STYLE('',(#311028));
#311028=SURFACE_STYLE_FILL_AREA(#311035);
#311035=FILL_AREA_STYLE('Opaque(122,133,145)',(#311042));
#311042=FILL_AREA_STYLE_COLOUR('Opaque(122,133,145)',#311049);
#311049=COLOUR_RGB('Opaque(122,133,145)',0.47843137254902,0.52156862745098,
0.568627450980392);
ENDSEC;
END-ISO-10303-21;
